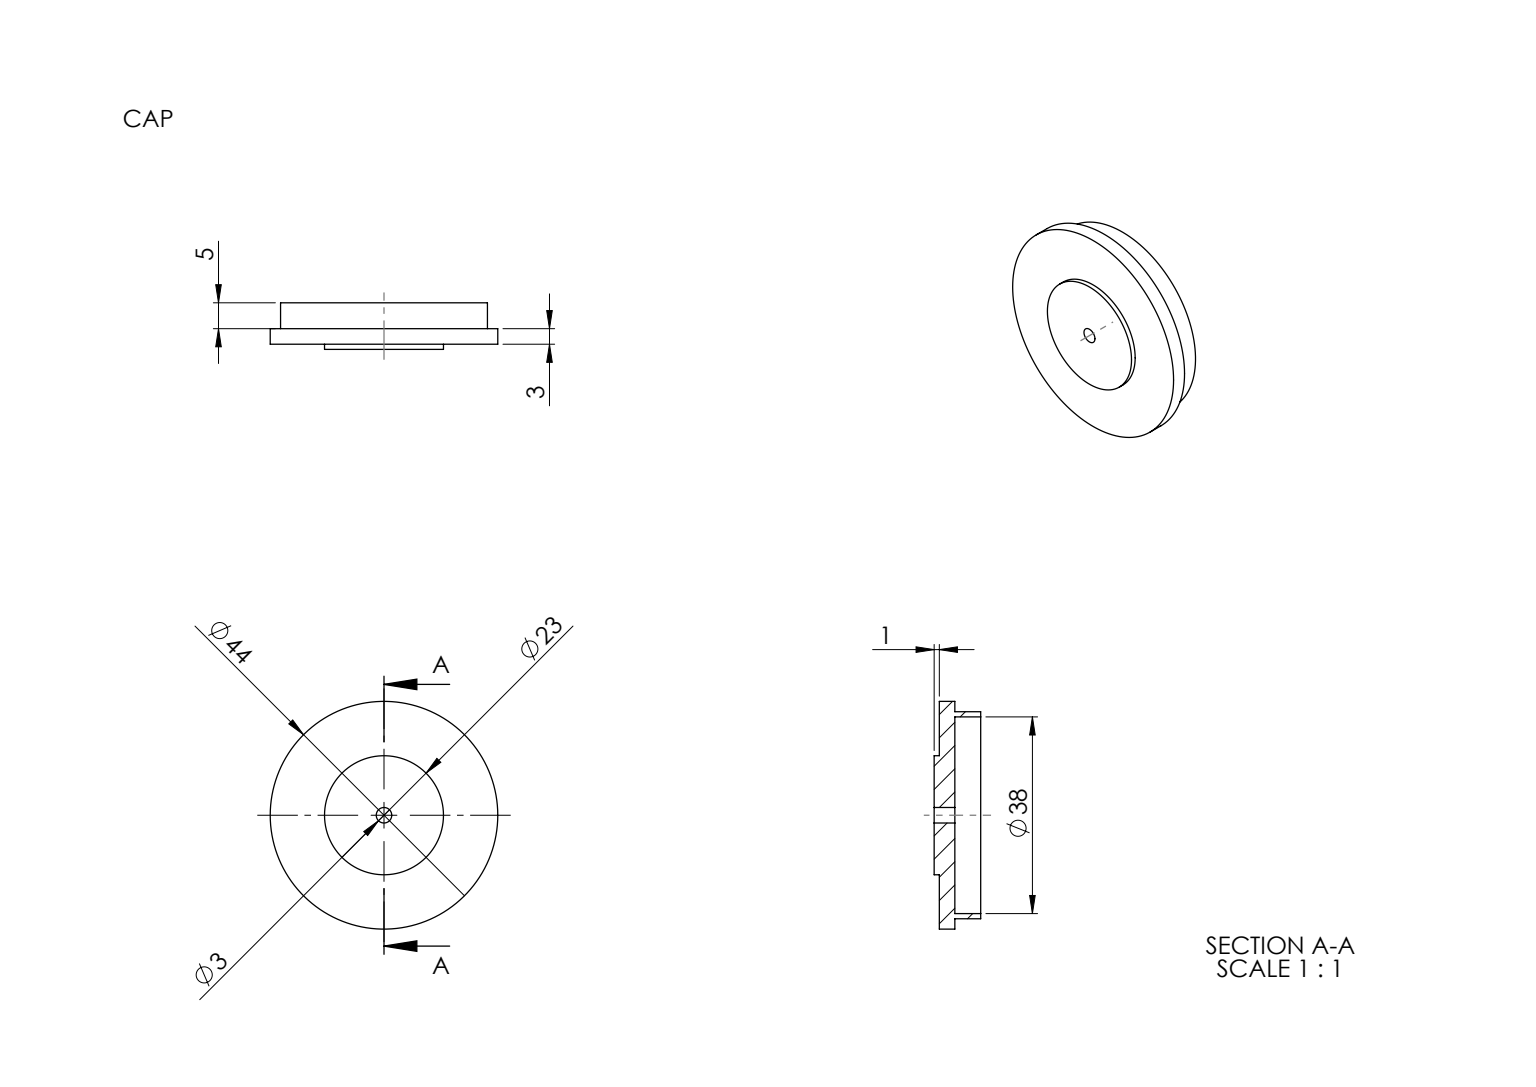
ISO-10303-21;
HEADER;
FILE_DESCRIPTION (('STEP AP214'),
    '1' );
FILE_NAME ('cap.step',
    '2026-10-08T12:30:53',
    ( '' ),
    ( '' ),
    'SwSTEP 2.0',
    'SolidWorks 2026',
    '' );
FILE_SCHEMA (( 'AUTOMOTIVE_DESIGN' ));
ENDSEC;

DATA;
#14=CARTESIAN_POINT ( 'NONE',  ( -22.00000000000000000, 0.000000000000000000, 3.000000000000000000 ) ) ;
#15=EDGE_CURVE ( 'NONE', #3183, #6148, #9804, .T. ) ;
#25=LINE ( 'NONE', #9459, #11094 ) ;
#162=CARTESIAN_POINT ( 'NONE',  ( 0.000000000000000000, 0.000000000000000000, -5.000000000000000000 ) ) ;
#181=ORIENTED_EDGE ( 'NONE', *, *, #10463, .F. ) ;
#186=CIRCLE ( 'NONE', #2152, 19.00000000000000000 ) ;
#188=SURFACE_STYLE_USAGE ( .BOTH. , #11225 ) ;
#197=( GEOMETRIC_REPRESENTATION_CONTEXT ( 3 ) GLOBAL_UNCERTAINTY_ASSIGNED_CONTEXT ( ( #10141 ) ) GLOBAL_UNIT_ASSIGNED_CONTEXT ( ( #1001, #11583, #11461 ) ) REPRESENTATION_CONTEXT ( 'NONE', 'WORKASPACE' ) );
#231=ORIENTED_EDGE ( 'NONE', *, *, #8776, .T. ) ;
#361=EDGE_CURVE ( 'NONE', #5937, #3303, #11757, .T. ) ;
#363=VERTEX_POINT ( 'NONE', #2521 ) ;
#403=CARTESIAN_POINT ( 'NONE',  ( 1.500000000000000222, 0.000000000000000000, 0.000000000000000000 ) ) ;
#426=EDGE_LOOP ( 'NONE', ( #4660, #3753, #2493, #2371 ) ) ;
#451=AXIS2_PLACEMENT_3D ( 'NONE', #7259, #6360, #5257 ) ;
#452=DIRECTION ( 'NONE',  ( 0.000000000000000000, 0.000000000000000000, 1.000000000000000000 ) ) ;
#519=EDGE_LOOP ( 'NONE', ( #2423, #3597, #5919, #11454 ) ) ;
#553=AXIS2_PLACEMENT_3D ( 'NONE', #11181, #7367, #11111 ) ;
#570=CARTESIAN_POINT ( 'NONE',  ( 0.000000000000000000, 0.000000000000000000, 0.000000000000000000 ) ) ;
#579=ORIENTED_EDGE ( 'NONE', *, *, #12044, .T. ) ;
#659=EDGE_LOOP ( 'NONE', ( #6044, #5887 ) ) ;
#704=EDGE_LOOP ( 'NONE', ( #4877, #4210, #1502, #2089 ) ) ;
#713=VECTOR ( 'NONE', #3546, 1000.000000000000000 ) ;
#761=ORIENTED_EDGE ( 'NONE', *, *, #7434, .T. ) ;
#786=DIRECTION ( 'NONE',  ( 0.000000000000000000, 0.000000000000000000, -1.000000000000000000 ) ) ;
#799=STYLED_ITEM ( 'NONE', ( #10298 ), #8499 ) ;
#870=CYLINDRICAL_SURFACE ( 'NONE', #2804, 11.50000000000000178 ) ;
#876=DIRECTION ( 'NONE',  ( 0.000000000000000000, 0.000000000000000000, 1.000000000000000000 ) ) ;
#890=ORIENTED_EDGE ( 'NONE', *, *, #7426, .T. ) ;
#917=ORIENTED_EDGE ( 'NONE', *, *, #10322, .F. ) ;
#937=CARTESIAN_POINT ( 'NONE',  ( 0.000000000000000000, 0.000000000000000000, -5.000000000000000000 ) ) ;
#1001=( LENGTH_UNIT ( ) NAMED_UNIT ( * ) SI_UNIT ( .MILLI., .METRE. ) );
#1016=CLOSED_SHELL ( 'NONE', ( #10067, #9974, #10631, #10029, #1210, #9209, #4991, #9798, #10209, #9430, #5118, #1787, #6730, #10852, #7083 ) ) ;
#1027=CARTESIAN_POINT ( 'NONE',  ( 0.000000000000000000, 0.000000000000000000, 3.000000000000000000 ) ) ;
#1071=CARTESIAN_POINT ( 'NONE',  ( 0.000000000000000000, 0.000000000000000000, 0.000000000000000000 ) ) ;
#1117=FILL_AREA_STYLE ('',( #2038 ) ) ;
#1138=APPLICATION_CONTEXT ( 'automotive_design' ) ;
#1163=DIRECTION ( 'NONE',  ( 1.000000000000000000, 0.000000000000000000, -0.000000000000000000 ) ) ;
#1175=SHAPE_REPRESENTATION_RELATIONSHIP ( 'NONE' , 'NONE' ,  #6315, #8499 ) ;
#1210=ADVANCED_FACE ( 'NONE', ( #10682 ), #1315, .T. ) ;
#1246=FACE_OUTER_BOUND ( 'NONE', #3018, .T. ) ;
#1263=DIRECTION ( 'NONE',  ( -0.000000000000000000, -0.000000000000000000, -1.000000000000000000 ) ) ;
#1315=CYLINDRICAL_SURFACE ( 'NONE', #2574, 22.00000000000000000 ) ;
#1336=UNCERTAINTY_MEASURE_WITH_UNIT (LENGTH_MEASURE( 1.000000000000000082E-05 ), #7812, 'distance_accuracy_value', 'NONE');
#1447=FILL_AREA_STYLE ('',( #1505 ) ) ;
#1462=UNCERTAINTY_MEASURE_WITH_UNIT (LENGTH_MEASURE( 1.000000000000000082E-05 ), #12067, 'distance_accuracy_value', 'NONE');
#1468=VERTEX_POINT ( 'NONE', #14 ) ;
#1478=EDGE_LOOP ( 'NONE', ( #12078, #1615, #9783, #231 ) ) ;
#1502=ORIENTED_EDGE ( 'NONE', *, *, #4060, .T. ) ;
#1505=FILL_AREA_STYLE_COLOUR ( '', #10720 ) ;
#1530=ORIENTED_EDGE ( 'NONE', *, *, #2012, .T. ) ;
#1551=DIRECTION ( 'NONE',  ( 0.000000000000000000, 0.000000000000000000, 1.000000000000000000 ) ) ;
#1554=CARTESIAN_POINT ( 'NONE',  ( 0.000000000000000000, 0.000000000000000000, -5.000000000000000000 ) ) ;
#1570=AXIS2_PLACEMENT_3D ( 'NONE', #8663, #2226, #11525 ) ;
#1603=ORIENTED_EDGE ( 'NONE', *, *, #11072, .T. ) ;
#1613=DIRECTION ( 'NONE',  ( -1.000000000000000000, 0.000000000000000000, 0.000000000000000000 ) ) ;
#1615=ORIENTED_EDGE ( 'NONE', *, *, #6080, .F. ) ;
#1640=VERTEX_POINT ( 'NONE', #4561 ) ;
#1660=ORIENTED_EDGE ( 'NONE', *, *, #8034, .T. ) ;
#1674=CARTESIAN_POINT ( 'NONE',  ( 0.000000000000000000, 0.000000000000000000, 0.000000000000000000 ) ) ;
#1724=EDGE_CURVE ( 'NONE', #9035, #12008, #3917, .T. ) ;
#1743=CARTESIAN_POINT ( 'NONE',  ( -19.00000000000000000, 2.326828918379970970E-15, -5.000000000000000000 ) ) ;
#1777=DIRECTION ( 'NONE',  ( -1.000000000000000000, 0.000000000000000000, 0.000000000000000000 ) ) ;
#1787=ADVANCED_FACE ( 'NONE', ( #7671 ), #2283, .F. ) ;
#1818=AXIS2_PLACEMENT_3D ( 'NONE', #4837, #7582, #2884 ) ;
#1852=EDGE_LOOP ( 'NONE', ( #10136, #1603, #7225, #5129 ) ) ;
#1854=ORIENTED_EDGE ( 'NONE', *, *, #10659, .F. ) ;
#1961=DIRECTION ( 'NONE',  ( -0.000000000000000000, -0.000000000000000000, -1.000000000000000000 ) ) ;
#1987=AXIS2_PLACEMENT_3D ( 'NONE', #5912, #3331, #8784 ) ;
#2012=EDGE_CURVE ( 'NONE', #5418, #3455, #8821, .T. ) ;
#2031=ORIENTED_EDGE ( 'NONE', *, *, #7774, .F. ) ;
#2033=LINE ( 'NONE', #3196, #3330 ) ;
#2038=FILL_AREA_STYLE_COLOUR ( '', #9398 ) ;
#2083=DIRECTION ( 'NONE',  ( 0.000000000000000000, 0.000000000000000000, 1.000000000000000000 ) ) ;
#2089=ORIENTED_EDGE ( 'NONE', *, *, #7426, .F. ) ;
#2118=CARTESIAN_POINT ( 'NONE',  ( 22.00000000000000000, 2.694222958124176809E-15, 0.000000000000000000 ) ) ;
#2129=EDGE_LOOP ( 'NONE', ( #4383, #10291 ) ) ;
#2152=AXIS2_PLACEMENT_3D ( 'NONE', #4061, #3263, #1613 ) ;
#2187=CARTESIAN_POINT ( 'NONE',  ( 20.00000000000000000, 0.000000000000000000, -5.000000000000000000 ) ) ;
#2191=DIRECTION ( 'NONE',  ( 0.000000000000000000, 0.000000000000000000, -1.000000000000000000 ) ) ;
#2226=DIRECTION ( 'NONE',  ( 0.000000000000000000, 0.000000000000000000, 1.000000000000000000 ) ) ;
#2238=ORIENTED_EDGE ( 'NONE', *, *, #2480, .T. ) ;
#2262=FACE_OUTER_BOUND ( 'NONE', #3512, .T. ) ;
#2264=AXIS2_PLACEMENT_3D ( 'NONE', #937, #4231, #2334 ) ;
#2283=CYLINDRICAL_SURFACE ( 'NONE', #7028, 1.500000000000000222 ) ;
#2293=LINE ( 'NONE', #3163, #10586 ) ;
#2294=CARTESIAN_POINT ( 'NONE',  ( 0.000000000000000000, 0.000000000000000000, 3.000000000000000000 ) ) ;
#2297=AXIS2_PLACEMENT_3D ( 'NONE', #570, #452, #6089 ) ;
#2311=VECTOR ( 'NONE', #5927, 1000.000000000000000 ) ;
#2312=EDGE_CURVE ( 'NONE', #10264, #11249, #10004, .T. ) ;
#2334=DIRECTION ( 'NONE',  ( -1.000000000000000000, 0.000000000000000000, -0.000000000000000000 ) ) ;
#2348=PLANE ( 'NONE',  #2297 ) ;
#2371=ORIENTED_EDGE ( 'NONE', *, *, #2312, .T. ) ;
#2378=AXIS2_PLACEMENT_3D ( 'NONE', #4592, #7205, #2817 ) ;
#2386=AXIS2_PLACEMENT_3D ( 'NONE', #2761, #8577, #7583 ) ;
#2413=CARTESIAN_POINT ( 'NONE',  ( -1.500000000000000222, 1.836970198721030181E-16, 0.000000000000000000 ) ) ;
#2423=ORIENTED_EDGE ( 'NONE', *, *, #6105, .F. ) ;
#2456=CARTESIAN_POINT ( 'NONE',  ( 19.00000000000000000, 0.000000000000000000, 0.000000000000000000 ) ) ;
#2465=EDGE_CURVE ( 'NONE', #7274, #2665, #9618, .T. ) ;
#2480=EDGE_CURVE ( 'NONE', #11249, #10264, #5905, .T. ) ;
#2492=ORIENTED_EDGE ( 'NONE', *, *, #9536, .F. ) ;
#2493=ORIENTED_EDGE ( 'NONE', *, *, #7774, .T. ) ;
#2521=CARTESIAN_POINT ( 'NONE',  ( -19.00000000000000000, 2.326828918379970970E-15, 0.000000000000000000 ) ) ;
#2574=AXIS2_PLACEMENT_3D ( 'NONE', #2294, #4139, #3044 ) ;
#2618=ORIENTED_EDGE ( 'NONE', *, *, #9536, .T. ) ;
#2630=EDGE_CURVE ( 'NONE', #1468, #3303, #8690, .T. ) ;
#2638=ORIENTED_EDGE ( 'NONE', *, *, #6237, .T. ) ;
#2653=DIRECTION ( 'NONE',  ( 1.000000000000000000, 0.000000000000000000, 0.000000000000000000 ) ) ;
#2665=VERTEX_POINT ( 'NONE', #4713 ) ;
#2680=LINE ( 'NONE', #10945, #713 ) ;
#2761=CARTESIAN_POINT ( 'NONE',  ( 0.000000000000000000, 0.000000000000000000, 0.000000000000000000 ) ) ;
#2771=EDGE_CURVE ( 'NONE', #8914, #1640, #4882, .T. ) ;
#2804=AXIS2_PLACEMENT_3D ( 'NONE', #6668, #1961, #1777 ) ;
#2817=DIRECTION ( 'NONE',  ( 1.000000000000000000, 0.000000000000000000, 0.000000000000000000 ) ) ;
#2859=DIRECTION ( 'NONE',  ( 1.000000000000000000, 0.000000000000000000, 0.000000000000000000 ) ) ;
#2870=CARTESIAN_POINT ( 'NONE',  ( 0.000000000000000000, 0.000000000000000000, 0.000000000000000000 ) ) ;
#2883=ORIENTED_EDGE ( 'NONE', *, *, #6080, .T. ) ;
#2884=DIRECTION ( 'NONE',  ( 1.000000000000000000, 0.000000000000000000, 0.000000000000000000 ) ) ;
#2932=CARTESIAN_POINT ( 'NONE',  ( 0.000000000000000000, 0.000000000000000000, 4.000000000000000000 ) ) ;
#2959=MECHANICAL_DESIGN_GEOMETRIC_PRESENTATION_REPRESENTATION('',(#799),#197);
#2976=DIRECTION ( 'NONE',  ( 0.000000000000000000, 0.000000000000000000, 1.000000000000000000 ) ) ;
#3018=EDGE_LOOP ( 'NONE', ( #2883, #11867 ) ) ;
#3041=CARTESIAN_POINT ( 'NONE',  ( -11.50000000000000178, 0.000000000000000000, 3.000000000000000000 ) ) ;
#3044=DIRECTION ( 'NONE',  ( -1.000000000000000000, 0.000000000000000000, 0.000000000000000000 ) ) ;
#3062=DIRECTION ( 'NONE',  ( -0.000000000000000000, -0.000000000000000000, -1.000000000000000000 ) ) ;
#3084=CARTESIAN_POINT ( 'NONE',  ( 0.000000000000000000, 0.000000000000000000, -5.000000000000000000 ) ) ;
#3133=ORIENTED_EDGE ( 'NONE', *, *, #15, .F. ) ;
#3163=CARTESIAN_POINT ( 'NONE',  ( -11.50000000000000178, 0.000000000000000000, 4.000000000000000000 ) ) ;
#3183=VERTEX_POINT ( 'NONE', #9746 ) ;
#3196=CARTESIAN_POINT ( 'NONE',  ( -20.00000000000000000, 2.449293598294706513E-15, -5.000000000000000000 ) ) ;
#3263=DIRECTION ( 'NONE',  ( 0.000000000000000000, 0.000000000000000000, -1.000000000000000000 ) ) ;
#3300=EDGE_CURVE ( 'NONE', #9888, #363, #186, .T. ) ;
#3303=VERTEX_POINT ( 'NONE', #6261 ) ;
#3314=PLANE ( 'NONE',  #5235 ) ;
#3330=VECTOR ( 'NONE', #10473, 1000.000000000000000 ) ;
#3331=DIRECTION ( 'NONE',  ( 0.000000000000000000, 0.000000000000000000, -1.000000000000000000 ) ) ;
#3416=SURFACE_STYLE_USAGE ( .BOTH. , #4320 ) ;
#3426=ORIENTED_EDGE ( 'NONE', *, *, #361, .F. ) ;
#3455=VERTEX_POINT ( 'NONE', #7223 ) ;
#3470=ORIENTED_EDGE ( 'NONE', *, *, #2771, .T. ) ;
#3471=ORIENTED_EDGE ( 'NONE', *, *, #3300, .F. ) ;
#3512=EDGE_LOOP ( 'NONE', ( #11119, #3426 ) ) ;
#3519=DIRECTION ( 'NONE',  ( -0.000000000000000000, -0.000000000000000000, 1.000000000000000000 ) ) ;
#3543=CARTESIAN_POINT ( 'NONE',  ( 0.000000000000000000, 0.000000000000000000, 4.000000000000000000 ) ) ;
#3546=DIRECTION ( 'NONE',  ( -0.000000000000000000, -0.000000000000000000, 1.000000000000000000 ) ) ;
#3564=CIRCLE ( 'NONE', #2386, 1.500000000000000222 ) ;
#3597=ORIENTED_EDGE ( 'NONE', *, *, #2012, .F. ) ;
#3603=ORIENTED_EDGE ( 'NONE', *, *, #8034, .F. ) ;
#3621=ORIENTED_EDGE ( 'NONE', *, *, #11008, .F. ) ;
#3696=CYLINDRICAL_SURFACE ( 'NONE', #9852, 20.00000000000000000 ) ;
#3753=ORIENTED_EDGE ( 'NONE', *, *, #7434, .F. ) ;
#3754=EDGE_CURVE ( 'NONE', #3183, #11249, #2033, .T. ) ;
#3757=AXIS2_PLACEMENT_3D ( 'NONE', #5217, #4293, #11762 ) ;
#3760=AXIS2_PLACEMENT_3D ( 'NONE', #9170, #786, #6541 ) ;
#3833=DIRECTION ( 'NONE',  ( 1.000000000000000000, 0.000000000000000000, 0.000000000000000000 ) ) ;
#3880=DIRECTION ( 'NONE',  ( -0.000000000000000000, -0.000000000000000000, 1.000000000000000000 ) ) ;
#3892=CIRCLE ( 'NONE', #553, 1.500000000000000222 ) ;
#3917=CIRCLE ( 'NONE', #1570, 11.50000000000000178 ) ;
#4060=EDGE_CURVE ( 'NONE', #2665, #7274, #11362, .T. ) ;
#4061=CARTESIAN_POINT ( 'NONE',  ( 0.000000000000000000, 0.000000000000000000, 0.000000000000000000 ) ) ;
#4139=DIRECTION ( 'NONE',  ( -0.000000000000000000, -0.000000000000000000, -1.000000000000000000 ) ) ;
#4210=ORIENTED_EDGE ( 'NONE', *, *, #10659, .T. ) ;
#4215=FACE_BOUND ( 'NONE', #10718, .T. ) ;
#4231=DIRECTION ( 'NONE',  ( 0.000000000000000000, 0.000000000000000000, -1.000000000000000000 ) ) ;
#4234=DIRECTION ( 'NONE',  ( 0.000000000000000000, 0.000000000000000000, 1.000000000000000000 ) ) ;
#4247=DIRECTION ( 'NONE',  ( -0.000000000000000000, -0.000000000000000000, 1.000000000000000000 ) ) ;
#4293=DIRECTION ( 'NONE',  ( 0.000000000000000000, 0.000000000000000000, 1.000000000000000000 ) ) ;
#4320=SURFACE_SIDE_STYLE ('',( #5182 ) ) ;
#4350=CIRCLE ( 'NONE', #7672, 22.00000000000000000 ) ;
#4360=AXIS2_PLACEMENT_3D ( 'NONE', #11569, #2083, #1163 ) ;
#4383=ORIENTED_EDGE ( 'NONE', *, *, #3300, .T. ) ;
#4438=EDGE_CURVE ( 'NONE', #5418, #9035, #2293, .T. ) ;
#4518=PLANE ( 'NONE',  #9168 ) ;
#4522=DIRECTION ( 'NONE',  ( -1.000000000000000000, 0.000000000000000000, 0.000000000000000000 ) ) ;
#4553=CIRCLE ( 'NONE', #11389, 11.50000000000000178 ) ;
#4561=CARTESIAN_POINT ( 'NONE',  ( 19.00000000000000000, 0.000000000000000000, -5.000000000000000000 ) ) ;
#4592=CARTESIAN_POINT ( 'NONE',  ( 0.000000000000000000, 0.000000000000000000, 4.000000000000000000 ) ) ;
#4660=ORIENTED_EDGE ( 'NONE', *, *, #3754, .F. ) ;
#4698=ORIENTED_EDGE ( 'NONE', *, *, #15, .T. ) ;
#4713=CARTESIAN_POINT ( 'NONE',  ( -1.500000000000000222, 1.836970198721030181E-16, 4.000000000000000000 ) ) ;
#4769=DIRECTION ( 'NONE',  ( 1.000000000000000000, 0.000000000000000000, 0.000000000000000000 ) ) ;
#4771=DIRECTION ( 'NONE',  ( -1.000000000000000000, 0.000000000000000000, 0.000000000000000000 ) ) ;
#4778=CYLINDRICAL_SURFACE ( 'NONE', #9112, 19.00000000000000000 ) ;
#4837=CARTESIAN_POINT ( 'NONE',  ( 0.000000000000000000, 0.000000000000000000, -5.000000000000000000 ) ) ;
#4852=LINE ( 'NONE', #8350, #6023 ) ;
#4866=LINE ( 'NONE', #8604, #5000 ) ;
#4877=ORIENTED_EDGE ( 'NONE', *, *, #11554, .F. ) ;
#4882=CIRCLE ( 'NONE', #5463, 19.00000000000000000 ) ;
#4902=( GEOMETRIC_REPRESENTATION_CONTEXT ( 3 ) GLOBAL_UNCERTAINTY_ASSIGNED_CONTEXT ( ( #1462 ) ) GLOBAL_UNIT_ASSIGNED_CONTEXT ( ( #12067, #11284, #11162 ) ) REPRESENTATION_CONTEXT ( 'NONE', 'WORKASPACE' ) );
#4919=CARTESIAN_POINT ( 'NONE',  ( 22.00000000000000000, 2.694222958124176809E-15, 3.000000000000000000 ) ) ;
#4991=ADVANCED_FACE ( 'NONE', ( #7761 ), #11500, .T. ) ;
#5000=VECTOR ( 'NONE', #7108, 1000.000000000000000 ) ;
#5010=VERTEX_POINT ( 'NONE', #5876 ) ;
#5036=AXIS2_PLACEMENT_3D ( 'NONE', #11948, #8287, #12013 ) ;
#5059=PRESENTATION_STYLE_ASSIGNMENT (( #3416 ) ) ;
#5077=ORIENTED_EDGE ( 'NONE', *, *, #11554, .T. ) ;
#5113=EDGE_LOOP ( 'NONE', ( #1854, #3603, #890, #7593 ) ) ;
#5118=ADVANCED_FACE ( 'NONE', ( #4215, #11978 ), #4518, .T. ) ;
#5121=DIRECTION ( 'NONE',  ( 1.000000000000000000, 0.000000000000000000, 0.000000000000000000 ) ) ;
#5129=ORIENTED_EDGE ( 'NONE', *, *, #2630, .F. ) ;
#5182=SURFACE_STYLE_FILL_AREA ( #1447 ) ;
#5217=CARTESIAN_POINT ( 'NONE',  ( 0.000000000000000000, 0.000000000000000000, 0.000000000000000000 ) ) ;
#5233=CIRCLE ( 'NONE', #9530, 22.00000000000000000 ) ;
#5235=AXIS2_PLACEMENT_3D ( 'NONE', #8891, #4234, #7959 ) ;
#5257=DIRECTION ( 'NONE',  ( -1.000000000000000000, 0.000000000000000000, 0.000000000000000000 ) ) ;
#5294=PRODUCT_DEFINITION_FORMATION_WITH_SPECIFIED_SOURCE ( 'ANY', '', #11573, .NOT_KNOWN. ) ;
#5418=VERTEX_POINT ( 'NONE', #5561 ) ;
#5463=AXIS2_PLACEMENT_3D ( 'NONE', #162, #2191, #4771 ) ;
#5519=CARTESIAN_POINT ( 'NONE',  ( 0.000000000000000000, 0.000000000000000000, -5.000000000000000000 ) ) ;
#5561=CARTESIAN_POINT ( 'NONE',  ( -11.50000000000000178, 0.000000000000000000, 4.000000000000000000 ) ) ;
#5573=ORIENTED_EDGE ( 'NONE', *, *, #4060, .F. ) ;
#5591=PLANE ( 'NONE',  #2264 ) ;
#5609=DIRECTION ( 'NONE',  ( 1.000000000000000000, 0.000000000000000000, 0.000000000000000000 ) ) ;
#5628=CARTESIAN_POINT ( 'NONE',  ( 0.000000000000000000, 0.000000000000000000, 4.000000000000000000 ) ) ;
#5650=FACE_OUTER_BOUND ( 'NONE', #9973, .T. ) ;
#5691=CARTESIAN_POINT ( 'NONE',  ( -22.00000000000000000, 0.000000000000000000, 3.000000000000000000 ) ) ;
#5703=DIRECTION ( 'NONE',  ( 1.000000000000000000, 0.000000000000000000, 0.000000000000000000 ) ) ;
#5763=FACE_OUTER_BOUND ( 'NONE', #10094, .T. ) ;
#5876=CARTESIAN_POINT ( 'NONE',  ( -1.500000000000000222, 1.836970198721030181E-16, 0.000000000000000000 ) ) ;
#5887=ORIENTED_EDGE ( 'NONE', *, *, #2480, .F. ) ;
#5905=CIRCLE ( 'NONE', #3760, 20.00000000000000000 ) ;
#5912=CARTESIAN_POINT ( 'NONE',  ( 0.000000000000000000, 0.000000000000000000, -5.000000000000000000 ) ) ;
#5919=ORIENTED_EDGE ( 'NONE', *, *, #4438, .T. ) ;
#5927=DIRECTION ( 'NONE',  ( -0.000000000000000000, -0.000000000000000000, 1.000000000000000000 ) ) ;
#5937=VERTEX_POINT ( 'NONE', #2118 ) ;
#5944=PLANE ( 'NONE',  #4360 ) ;
#6023=VECTOR ( 'NONE', #8479, 1000.000000000000000 ) ;
#6036=( NAMED_UNIT ( * ) PLANE_ANGLE_UNIT ( ) SI_UNIT ( $, .RADIAN. ) );
#6044=ORIENTED_EDGE ( 'NONE', *, *, #2312, .F. ) ;
#6060=EDGE_LOOP ( 'NONE', ( #9184, #2638, #3471, #2492 ) ) ;
#6080=EDGE_CURVE ( 'NONE', #1468, #10781, #5233, .T. ) ;
#6089=DIRECTION ( 'NONE',  ( 1.000000000000000000, 0.000000000000000000, -0.000000000000000000 ) ) ;
#6105=EDGE_CURVE ( 'NONE', #3455, #12008, #25, .T. ) ;
#6141=VECTOR ( 'NONE', #9821, 1000.000000000000000 ) ;
#6148=VERTEX_POINT ( 'NONE', #6575 ) ;
#6207=CYLINDRICAL_SURFACE ( 'NONE', #5036, 11.50000000000000178 ) ;
#6237=EDGE_CURVE ( 'NONE', #8914, #363, #4866, .T. ) ;
#6239=ORIENTED_EDGE ( 'NONE', *, *, #12044, .F. ) ;
#6261=CARTESIAN_POINT ( 'NONE',  ( -22.00000000000000000, 0.000000000000000000, 0.000000000000000000 ) ) ;
#6315=SHAPE_REPRESENTATION ( 'cap', ( #8474 ), #4902 ) ;
#6360=DIRECTION ( 'NONE',  ( 0.000000000000000000, 0.000000000000000000, -1.000000000000000000 ) ) ;
#6381=ORIENTED_EDGE ( 'NONE', *, *, #6237, .F. ) ;
#6396=ORIENTED_EDGE ( 'NONE', *, *, #2771, .F. ) ;
#6506=FACE_BOUND ( 'NONE', #6950, .T. ) ;
#6541=DIRECTION ( 'NONE',  ( -1.000000000000000000, 0.000000000000000000, 0.000000000000000000 ) ) ;
#6563=SURFACE_STYLE_FILL_AREA ( #1117 ) ;
#6575=CARTESIAN_POINT ( 'NONE',  ( 20.00000000000000000, 0.000000000000000000, -5.000000000000000000 ) ) ;
#6593=DIRECTION ( 'NONE',  ( 0.000000000000000000, 0.000000000000000000, 1.000000000000000000 ) ) ;
#6668=CARTESIAN_POINT ( 'NONE',  ( 0.000000000000000000, 0.000000000000000000, 4.000000000000000000 ) ) ;
#6730=ADVANCED_FACE ( 'NONE', ( #5650, #6506 ), #5591, .T. ) ;
#6745=DIRECTION ( 'NONE',  ( -1.000000000000000000, 0.000000000000000000, 0.000000000000000000 ) ) ;
#6763=APPLICATION_CONTEXT ( 'automotive_design' ) ;
#6801=AXIS2_PLACEMENT_3D ( 'NONE', #6944, #7876, #5121 ) ;
#6812=CARTESIAN_POINT ( 'NONE',  ( 0.000000000000000000, 0.000000000000000000, 3.000000000000000000 ) ) ;
#6850=AXIS2_PLACEMENT_3D ( 'NONE', #9255, #876, #8340 ) ;
#6932=LINE ( 'NONE', #2413, #6141 ) ;
#6944=CARTESIAN_POINT ( 'NONE',  ( 0.000000000000000000, 0.000000000000000000, 0.000000000000000000 ) ) ;
#6950=EDGE_LOOP ( 'NONE', ( #3621, #6396 ) ) ;
#6954=ORIENTED_EDGE ( 'NONE', *, *, #4438, .F. ) ;
#6989=FACE_OUTER_BOUND ( 'NONE', #2129, .T. ) ;
#7028=AXIS2_PLACEMENT_3D ( 'NONE', #1071, #3880, #7603 ) ;
#7056=EDGE_LOOP ( 'NONE', ( #1530, #9422 ) ) ;
#7076=PRODUCT_DEFINITION_CONTEXT ( 'detailed design', #1138, 'design' ) ;
#7083=ADVANCED_FACE ( 'NONE', ( #9307 ), #4778, .F. ) ;
#7089=CIRCLE ( 'NONE', #8677, 11.50000000000000178 ) ;
#7108=DIRECTION ( 'NONE',  ( -0.000000000000000000, -0.000000000000000000, 1.000000000000000000 ) ) ;
#7205=DIRECTION ( 'NONE',  ( 0.000000000000000000, 0.000000000000000000, 1.000000000000000000 ) ) ;
#7223=CARTESIAN_POINT ( 'NONE',  ( 11.50000000000000178, 1.408343819019456373E-15, 4.000000000000000000 ) ) ;
#7225=ORIENTED_EDGE ( 'NONE', *, *, #361, .T. ) ;
#7259=CARTESIAN_POINT ( 'NONE',  ( 0.000000000000000000, 0.000000000000000000, 0.000000000000000000 ) ) ;
#7274=VERTEX_POINT ( 'NONE', #8637 ) ;
#7367=DIRECTION ( 'NONE',  ( 0.000000000000000000, 0.000000000000000000, 1.000000000000000000 ) ) ;
#7390=MECHANICAL_DESIGN_GEOMETRIC_PRESENTATION_REPRESENTATION('',(#9152),#8771);
#7426=EDGE_CURVE ( 'NONE', #8709, #7274, #2680, .T. ) ;
#7434=EDGE_CURVE ( 'NONE', #6148, #3183, #10685, .T. ) ;
#7514=FACE_OUTER_BOUND ( 'NONE', #704, .T. ) ;
#7580=DIRECTION ( 'NONE',  ( -0.000000000000000000, -0.000000000000000000, 1.000000000000000000 ) ) ;
#7582=DIRECTION ( 'NONE',  ( -0.000000000000000000, -0.000000000000000000, 1.000000000000000000 ) ) ;
#7583=DIRECTION ( 'NONE',  ( 1.000000000000000000, 0.000000000000000000, 0.000000000000000000 ) ) ;
#7593=ORIENTED_EDGE ( 'NONE', *, *, #2465, .T. ) ;
#7603=DIRECTION ( 'NONE',  ( 1.000000000000000000, 0.000000000000000000, 0.000000000000000000 ) ) ;
#7629=VECTOR ( 'NONE', #8510, 1000.000000000000000 ) ;
#7671=FACE_OUTER_BOUND ( 'NONE', #5113, .T. ) ;
#7672=AXIS2_PLACEMENT_3D ( 'NONE', #1027, #9221, #2859 ) ;
#7750=PRODUCT_DEFINITION_SHAPE ( 'NONE', 'NONE',  #9427 ) ;
#7761=FACE_OUTER_BOUND ( 'NONE', #1478, .T. ) ;
#7774=EDGE_CURVE ( 'NONE', #6148, #10264, #10689, .T. ) ;
#7812=( LENGTH_UNIT ( ) NAMED_UNIT ( * ) SI_UNIT ( .MILLI., .METRE. ) );
#7864=FACE_BOUND ( 'NONE', #8112, .T. ) ;
#7876=DIRECTION ( 'NONE',  ( 0.000000000000000000, 0.000000000000000000, 1.000000000000000000 ) ) ;
#7889=CARTESIAN_POINT ( 'NONE',  ( 0.000000000000000000, 0.000000000000000000, 3.000000000000000000 ) ) ;
#7944=DIRECTION ( 'NONE',  ( -1.000000000000000000, 0.000000000000000000, 0.000000000000000000 ) ) ;
#7959=DIRECTION ( 'NONE',  ( 1.000000000000000000, 0.000000000000000000, -0.000000000000000000 ) ) ;
#7981=ORIENTED_EDGE ( 'NONE', *, *, #6105, .T. ) ;
#7985=( NAMED_UNIT ( * ) SI_UNIT ( $, .STERADIAN. ) SOLID_ANGLE_UNIT ( ) );
#8002=DIRECTION ( 'NONE',  ( 0.000000000000000000, 0.000000000000000000, -1.000000000000000000 ) ) ;
#8034=EDGE_CURVE ( 'NONE', #8709, #5010, #3892, .T. ) ;
#8078=CARTESIAN_POINT ( 'NONE',  ( 0.000000000000000000, 0.000000000000000000, 0.000000000000000000 ) ) ;
#8081=CIRCLE ( 'NONE', #451, 19.00000000000000000 ) ;
#8112=EDGE_LOOP ( 'NONE', ( #1660, #5077 ) ) ;
#8198=DIRECTION ( 'NONE',  ( 0.000000000000000000, 0.000000000000000000, 1.000000000000000000 ) ) ;
#8287=DIRECTION ( 'NONE',  ( -0.000000000000000000, -0.000000000000000000, -1.000000000000000000 ) ) ;
#8296=AXIS2_PLACEMENT_3D ( 'NONE', #3084, #10244, #6745 ) ;
#8335=FACE_OUTER_BOUND ( 'NONE', #6060, .T. ) ;
#8340=DIRECTION ( 'NONE',  ( 1.000000000000000000, 0.000000000000000000, 0.000000000000000000 ) ) ;
#8350=CARTESIAN_POINT ( 'NONE',  ( 19.00000000000000000, 0.000000000000000000, -5.000000000000000000 ) ) ;
#8365=DIRECTION ( 'NONE',  ( 0.000000000000000000, 0.000000000000000000, 1.000000000000000000 ) ) ;
#8474=AXIS2_PLACEMENT_3D ( 'NONE', #1674, #1551, #2653 ) ;
#8479=DIRECTION ( 'NONE',  ( -0.000000000000000000, -0.000000000000000000, 1.000000000000000000 ) ) ;
#8499=ADVANCED_BREP_SHAPE_REPRESENTATION ( '', ( #8710, #8474 ), #4902 ) ;
#8510=DIRECTION ( 'NONE',  ( -0.000000000000000000, -0.000000000000000000, -1.000000000000000000 ) ) ;
#8516=DIRECTION ( 'NONE',  ( 1.000000000000000000, 0.000000000000000000, 0.000000000000000000 ) ) ;
#8545=AXIS2_PLACEMENT_3D ( 'NONE', #11740, #8002, #4522 ) ;
#8562=DIRECTION ( 'NONE',  ( 1.000000000000000000, 0.000000000000000000, 0.000000000000000000 ) ) ;
#8577=DIRECTION ( 'NONE',  ( 0.000000000000000000, 0.000000000000000000, 1.000000000000000000 ) ) ;
#8604=CARTESIAN_POINT ( 'NONE',  ( -19.00000000000000000, 2.326828918379970970E-15, -5.000000000000000000 ) ) ;
#8623=CARTESIAN_POINT ( 'NONE',  ( 22.00000000000000000, 2.694222958124176809E-15, 3.000000000000000000 ) ) ;
#8637=CARTESIAN_POINT ( 'NONE',  ( 1.500000000000000222, 0.000000000000000000, 4.000000000000000000 ) ) ;
#8659=DIRECTION ( 'NONE',  ( -0.000000000000000000, -0.000000000000000000, -1.000000000000000000 ) ) ;
#8663=CARTESIAN_POINT ( 'NONE',  ( 0.000000000000000000, 0.000000000000000000, 3.000000000000000000 ) ) ;
#8677=AXIS2_PLACEMENT_3D ( 'NONE', #2932, #6593, #4769 ) ;
#8690=LINE ( 'NONE', #5691, #7629 ) ;
#8709=VERTEX_POINT ( 'NONE', #403 ) ;
#8710=MANIFOLD_SOLID_BREP ( 'Extrude-Thin1', #1016 ) ;
#8771=( GEOMETRIC_REPRESENTATION_CONTEXT ( 3 ) GLOBAL_UNCERTAINTY_ASSIGNED_CONTEXT ( ( #1336 ) ) GLOBAL_UNIT_ASSIGNED_CONTEXT ( ( #7812, #6036, #7985 ) ) REPRESENTATION_CONTEXT ( 'NONE', 'WORKASPACE' ) );
#8776=EDGE_CURVE ( 'NONE', #3303, #5937, #11885, .T. ) ;
#8784=DIRECTION ( 'NONE',  ( -1.000000000000000000, 0.000000000000000000, 0.000000000000000000 ) ) ;
#8821=CIRCLE ( 'NONE', #6850, 11.50000000000000178 ) ;
#8876=CIRCLE ( 'NONE', #8296, 19.00000000000000000 ) ;
#8879=FACE_BOUND ( 'NONE', #659, .T. ) ;
#8891=CARTESIAN_POINT ( 'NONE',  ( 0.000000000000000000, 0.000000000000000000, 3.000000000000000000 ) ) ;
#8914=VERTEX_POINT ( 'NONE', #1743 ) ;
#8968=ORIENTED_EDGE ( 'NONE', *, *, #3754, .T. ) ;
#9027=FACE_OUTER_BOUND ( 'NONE', #519, .T. ) ;
#9035=VERTEX_POINT ( 'NONE', #3041 ) ;
#9112=AXIS2_PLACEMENT_3D ( 'NONE', #9485, #7580, #8516 ) ;
#9152=STYLED_ITEM ( 'NONE', ( #5059 ), #8710 ) ;
#9168=AXIS2_PLACEMENT_3D ( 'NONE', #3543, #11854, #10829 ) ;
#9170=CARTESIAN_POINT ( 'NONE',  ( 0.000000000000000000, 0.000000000000000000, 0.000000000000000000 ) ) ;
#9184=ORIENTED_EDGE ( 'NONE', *, *, #11008, .T. ) ;
#9209=ADVANCED_FACE ( 'NONE', ( #7864, #6989 ), #2348, .F. ) ;
#9221=DIRECTION ( 'NONE',  ( 0.000000000000000000, 0.000000000000000000, 1.000000000000000000 ) ) ;
#9255=CARTESIAN_POINT ( 'NONE',  ( 0.000000000000000000, 0.000000000000000000, 4.000000000000000000 ) ) ;
#9307=FACE_OUTER_BOUND ( 'NONE', #11077, .T. ) ;
#9362=DIRECTION ( 'NONE',  ( 1.000000000000000000, 0.000000000000000000, 0.000000000000000000 ) ) ;
#9369=FACE_OUTER_BOUND ( 'NONE', #10694, .T. ) ;
#9398=COLOUR_RGB ( '', 0.08235294, 0.09019608, 0.10196078) ;
#9405=AXIS2_PLACEMENT_3D ( 'NONE', #5628, #8198, #9362 ) ;
#9422=ORIENTED_EDGE ( 'NONE', *, *, #10463, .T. ) ;
#9427=PRODUCT_DEFINITION ( 'UNKNOWN', '', #5294, #7076 ) ;
#9430=ADVANCED_FACE ( 'NONE', ( #9027 ), #6207, .T. ) ;
#9459=CARTESIAN_POINT ( 'NONE',  ( 11.50000000000000178, 1.408343819019456373E-15, 4.000000000000000000 ) ) ;
#9485=CARTESIAN_POINT ( 'NONE',  ( 0.000000000000000000, 0.000000000000000000, -5.000000000000000000 ) ) ;
#9503=LINE ( 'NONE', #4919, #11423 ) ;
#9530=AXIS2_PLACEMENT_3D ( 'NONE', #6812, #2976, #3833 ) ;
#9536=EDGE_CURVE ( 'NONE', #1640, #9888, #4852, .T. ) ;
#9577=DIRECTION ( 'NONE',  ( -0.000000000000000000, -0.000000000000000000, -1.000000000000000000 ) ) ;
#9618=CIRCLE ( 'NONE', #2378, 1.500000000000000222 ) ;
#9626=FACE_BOUND ( 'NONE', #9890, .T. ) ;
#9642=AXIS2_PLACEMENT_3D ( 'NONE', #7889, #3062, #7944 ) ;
#9656=AXIS2_PLACEMENT_3D ( 'NONE', #2870, #4247, #8562 ) ;
#9706=ORIENTED_EDGE ( 'NONE', *, *, #1724, .F. ) ;
#9730=DIRECTION ( 'NONE',  ( -1.000000000000000000, 0.000000000000000000, 0.000000000000000000 ) ) ;
#9746=CARTESIAN_POINT ( 'NONE',  ( -20.00000000000000000, 2.449293598294706513E-15, -5.000000000000000000 ) ) ;
#9783=ORIENTED_EDGE ( 'NONE', *, *, #2630, .T. ) ;
#9798=ADVANCED_FACE ( 'NONE', ( #9626, #1246 ), #3314, .T. ) ;
#9804=CIRCLE ( 'NONE', #1987, 20.00000000000000000 ) ;
#9821=DIRECTION ( 'NONE',  ( -0.000000000000000000, -0.000000000000000000, 1.000000000000000000 ) ) ;
#9852=AXIS2_PLACEMENT_3D ( 'NONE', #1554, #3519, #9997 ) ;
#9888=VERTEX_POINT ( 'NONE', #2456 ) ;
#9890=EDGE_LOOP ( 'NONE', ( #9706, #6239 ) ) ;
#9973=EDGE_LOOP ( 'NONE', ( #761, #4698 ) ) ;
#9974=ADVANCED_FACE ( 'NONE', ( #5763 ), #11325, .T. ) ;
#9997=DIRECTION ( 'NONE',  ( 1.000000000000000000, 0.000000000000000000, 0.000000000000000000 ) ) ;
#10004=CIRCLE ( 'NONE', #11575, 20.00000000000000000 ) ;
#10015=ORIENTED_EDGE ( 'NONE', *, *, #2465, .F. ) ;
#10029=ADVANCED_FACE ( 'NONE', ( #9369 ), #870, .T. ) ;
#10067=ADVANCED_FACE ( 'NONE', ( #8335 ), #12056, .F. ) ;
#10094=EDGE_LOOP ( 'NONE', ( #3133, #8968, #2238, #2031 ) ) ;
#10136=ORIENTED_EDGE ( 'NONE', *, *, #10575, .F. ) ;
#10141=UNCERTAINTY_MEASURE_WITH_UNIT (LENGTH_MEASURE( 1.000000000000000082E-05 ), #1001, 'distance_accuracy_value', 'NONE');
#10209=ADVANCED_FACE ( 'NONE', ( #8879, #2262 ), #5944, .F. ) ;
#10244=DIRECTION ( 'NONE',  ( 0.000000000000000000, 0.000000000000000000, -1.000000000000000000 ) ) ;
#10264=VERTEX_POINT ( 'NONE', #10705 ) ;
#10291=ORIENTED_EDGE ( 'NONE', *, *, #10322, .T. ) ;
#10298=PRESENTATION_STYLE_ASSIGNMENT (( #188 ) ) ;
#10322=EDGE_CURVE ( 'NONE', #363, #9888, #8081, .T. ) ;
#10463=EDGE_CURVE ( 'NONE', #3455, #5418, #7089, .T. ) ;
#10473=DIRECTION ( 'NONE',  ( -0.000000000000000000, -0.000000000000000000, 1.000000000000000000 ) ) ;
#10538=CARTESIAN_POINT ( 'NONE',  ( -20.00000000000000000, 2.449293598294706513E-15, 0.000000000000000000 ) ) ;
#10575=EDGE_CURVE ( 'NONE', #10781, #1468, #4350, .T. ) ;
#10579=SHAPE_DEFINITION_REPRESENTATION ( #7750, #6315 ) ;
#10586=VECTOR ( 'NONE', #1263, 1000.000000000000000 ) ;
#10631=ADVANCED_FACE ( 'NONE', ( #7514 ), #11257, .F. ) ;
#10659=EDGE_CURVE ( 'NONE', #5010, #2665, #6932, .T. ) ;
#10682=FACE_OUTER_BOUND ( 'NONE', #1852, .T. ) ;
#10685=CIRCLE ( 'NONE', #8545, 20.00000000000000000 ) ;
#10689=LINE ( 'NONE', #2187, #2311 ) ;
#10694=EDGE_LOOP ( 'NONE', ( #181, #7981, #579, #6954 ) ) ;
#10705=CARTESIAN_POINT ( 'NONE',  ( 20.00000000000000000, 0.000000000000000000, 0.000000000000000000 ) ) ;
#10718=EDGE_LOOP ( 'NONE', ( #10015, #5573 ) ) ;
#10720=COLOUR_RGB ( '', 0.08235294, 0.09019608, 0.10196078) ;
#10781=VERTEX_POINT ( 'NONE', #8623 ) ;
#10829=DIRECTION ( 'NONE',  ( 1.000000000000000000, 0.000000000000000000, -0.000000000000000000 ) ) ;
#10836=DIRECTION ( 'NONE',  ( 0.000000000000000000, 0.000000000000000000, -1.000000000000000000 ) ) ;
#10852=ADVANCED_FACE ( 'NONE', ( #11045 ), #3696, .T. ) ;
#10945=CARTESIAN_POINT ( 'NONE',  ( 1.500000000000000222, 0.000000000000000000, 0.000000000000000000 ) ) ;
#10949=CARTESIAN_POINT ( 'NONE',  ( 11.50000000000000178, 1.408343819019456373E-15, 3.000000000000000000 ) ) ;
#11008=EDGE_CURVE ( 'NONE', #1640, #8914, #8876, .T. ) ;
#11045=FACE_OUTER_BOUND ( 'NONE', #426, .T. ) ;
#11072=EDGE_CURVE ( 'NONE', #10781, #5937, #9503, .T. ) ;
#11077=EDGE_LOOP ( 'NONE', ( #6381, #3470, #2618, #917 ) ) ;
#11094=VECTOR ( 'NONE', #9577, 1000.000000000000000 ) ;
#11111=DIRECTION ( 'NONE',  ( 1.000000000000000000, 0.000000000000000000, 0.000000000000000000 ) ) ;
#11119=ORIENTED_EDGE ( 'NONE', *, *, #8776, .F. ) ;
#11145=DIRECTION ( 'NONE',  ( -0.000000000000000000, -0.000000000000000000, 1.000000000000000000 ) ) ;
#11162=( NAMED_UNIT ( * ) SI_UNIT ( $, .STERADIAN. ) SOLID_ANGLE_UNIT ( ) );
#11181=CARTESIAN_POINT ( 'NONE',  ( 0.000000000000000000, 0.000000000000000000, 0.000000000000000000 ) ) ;
#11225=SURFACE_SIDE_STYLE ('',( #6563 ) ) ;
#11249=VERTEX_POINT ( 'NONE', #10538 ) ;
#11257=CYLINDRICAL_SURFACE ( 'NONE', #9656, 1.500000000000000222 ) ;
#11284=( NAMED_UNIT ( * ) PLANE_ANGLE_UNIT ( ) SI_UNIT ( $, .RADIAN. ) );
#11325=CYLINDRICAL_SURFACE ( 'NONE', #11400, 20.00000000000000000 ) ;
#11362=CIRCLE ( 'NONE', #9405, 1.500000000000000222 ) ;
#11389=AXIS2_PLACEMENT_3D ( 'NONE', #12089, #8365, #5609 ) ;
#11400=AXIS2_PLACEMENT_3D ( 'NONE', #5519, #11145, #5703 ) ;
#11423=VECTOR ( 'NONE', #8659, 1000.000000000000000 ) ;
#11454=ORIENTED_EDGE ( 'NONE', *, *, #1724, .T. ) ;
#11461=( NAMED_UNIT ( * ) SI_UNIT ( $, .STERADIAN. ) SOLID_ANGLE_UNIT ( ) );
#11494=PRODUCT_CONTEXT ( 'NONE', #6763, 'mechanical' ) ;
#11500=CYLINDRICAL_SURFACE ( 'NONE', #9642, 22.00000000000000000 ) ;
#11525=DIRECTION ( 'NONE',  ( 1.000000000000000000, 0.000000000000000000, 0.000000000000000000 ) ) ;
#11554=EDGE_CURVE ( 'NONE', #5010, #8709, #3564, .T. ) ;
#11569=CARTESIAN_POINT ( 'NONE',  ( 0.000000000000000000, 0.000000000000000000, 0.000000000000000000 ) ) ;
#11573=PRODUCT ( 'cap', 'cap', '', ( #11494 ) ) ;
#11575=AXIS2_PLACEMENT_3D ( 'NONE', #8078, #10836, #9730 ) ;
#11583=( NAMED_UNIT ( * ) PLANE_ANGLE_UNIT ( ) SI_UNIT ( $, .RADIAN. ) );
#11740=CARTESIAN_POINT ( 'NONE',  ( 0.000000000000000000, 0.000000000000000000, -5.000000000000000000 ) ) ;
#11757=CIRCLE ( 'NONE', #3757, 22.00000000000000000 ) ;
#11762=DIRECTION ( 'NONE',  ( 1.000000000000000000, 0.000000000000000000, 0.000000000000000000 ) ) ;
#11854=DIRECTION ( 'NONE',  ( 0.000000000000000000, 0.000000000000000000, 1.000000000000000000 ) ) ;
#11867=ORIENTED_EDGE ( 'NONE', *, *, #10575, .T. ) ;
#11885=CIRCLE ( 'NONE', #6801, 22.00000000000000000 ) ;
#11948=CARTESIAN_POINT ( 'NONE',  ( 0.000000000000000000, 0.000000000000000000, 4.000000000000000000 ) ) ;
#11978=FACE_OUTER_BOUND ( 'NONE', #7056, .T. ) ;
#12008=VERTEX_POINT ( 'NONE', #10949 ) ;
#12013=DIRECTION ( 'NONE',  ( -1.000000000000000000, 0.000000000000000000, 0.000000000000000000 ) ) ;
#12044=EDGE_CURVE ( 'NONE', #12008, #9035, #4553, .T. ) ;
#12056=CYLINDRICAL_SURFACE ( 'NONE', #1818, 19.00000000000000000 ) ;
#12067=( LENGTH_UNIT ( ) NAMED_UNIT ( * ) SI_UNIT ( .MILLI., .METRE. ) );
#12078=ORIENTED_EDGE ( 'NONE', *, *, #11072, .F. ) ;
#12089=CARTESIAN_POINT ( 'NONE',  ( 0.000000000000000000, 0.000000000000000000, 3.000000000000000000 ) ) ;
ENDSEC;
END-ISO-10303-21;
